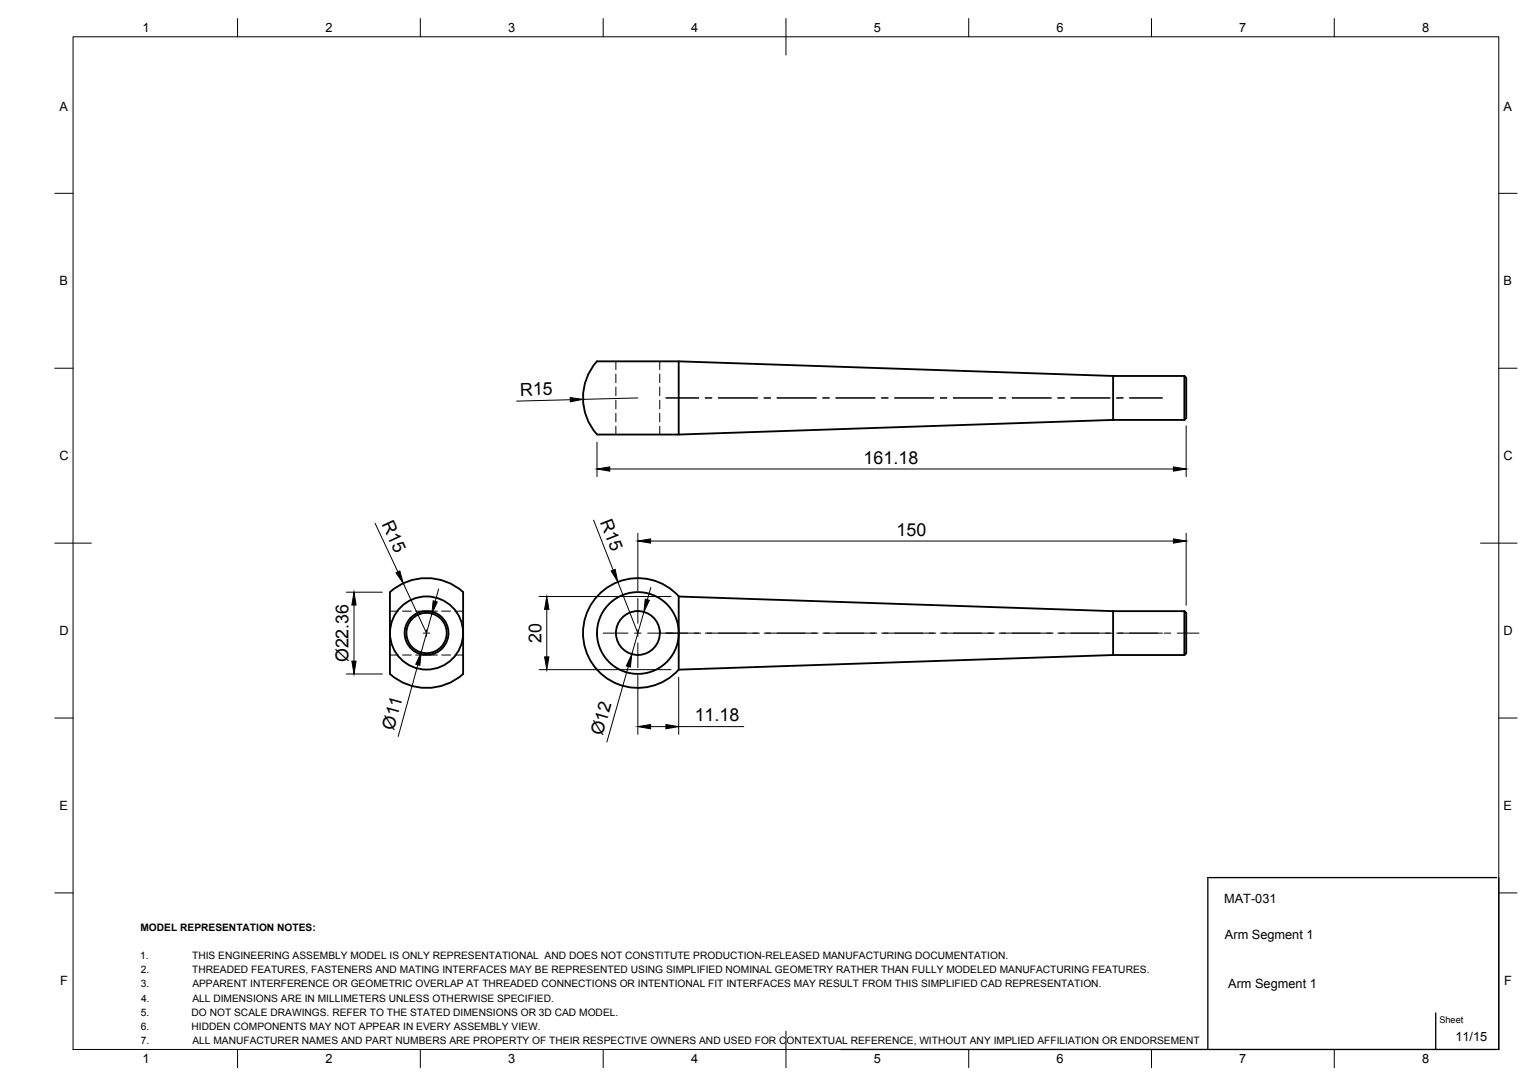
ISO-10303-21;
HEADER;
/* Generated by software containing ST-Developer
 * from STEP Tools, Inc. (www.steptools.com) 
 */

FILE_DESCRIPTION(
/* description */ ('STEP AP214'),
/* implementation_level */ '2;1');

FILE_NAME(
/* name */ 'Arm Segment 1.step',
/* time_stamp */ '2026-11-14T06:58:01-08:00',
/* author */ (''),
/* organization */ (''),
/* preprocessor_version */ 'ST-DEVELOPER v20.2',
/* originating_system */ 'Autodesk Translation Framework v15.17.0.0',
/* authorisation */ '');

FILE_SCHEMA (('AUTOMOTIVE_DESIGN { 1 0 10303 214 3 1 1 }'));
ENDSEC;

DATA;
#10=MECHANICAL_DESIGN_GEOMETRIC_PRESENTATION_REPRESENTATION('',(#1154),#38635);
#87=SPHERICAL_SURFACE('',#18128,15.);
#88=SPHERICAL_SURFACE('',#18136,15.);
#876=FACE_BOUND('',#2871,.T.);
#877=FACE_BOUND('',#2873,.T.);
#1027=CONICAL_SURFACE('',#18140,6.,0.0336517539394116);
#1028=CONICAL_SURFACE('',#18144,5.5,0.785398163397448);
#1120=SHAPE_REPRESENTATION_RELATIONSHIP('SRR','None',#38693,#1134);
#1134=ADVANCED_BREP_SHAPE_REPRESENTATION('',(#1180),#38629);
#1154=STYLED_ITEM('',(#38765),#1180);
#1180=MANIFOLD_SOLID_BREP('Body1',#17620);
#1260=PLANE('',#18146);
#1261=PLANE('',#18147);
#1262=PLANE('',#18148);
#1843=FACE_OUTER_BOUND('',#2863,.T.);
#1844=FACE_OUTER_BOUND('',#2864,.T.);
#1845=FACE_OUTER_BOUND('',#2865,.T.);
#1846=FACE_OUTER_BOUND('',#2866,.T.);
#1847=FACE_OUTER_BOUND('',#2867,.T.);
#1848=FACE_OUTER_BOUND('',#2868,.T.);
#1849=FACE_OUTER_BOUND('',#2869,.T.);
#1850=FACE_OUTER_BOUND('',#2870,.T.);
#1851=FACE_OUTER_BOUND('',#2872,.T.);
#2863=EDGE_LOOP('',(#11861,#11862,#11863,#11864));
#2864=EDGE_LOOP('',(#11865,#11866,#11867,#11868));
#2865=EDGE_LOOP('',(#11869,#11870,#11871,#11872));
#2866=EDGE_LOOP('',(#11873,#11874,#11875,#11876,#11877));
#2867=EDGE_LOOP('',(#11878,#11879,#11880,#11881));
#2868=EDGE_LOOP('',(#11882,#11883,#11884,#11885));
#2869=EDGE_LOOP('',(#11886));
#2870=EDGE_LOOP('',(#11887,#11888));
#2871=EDGE_LOOP('',(#11889));
#2872=EDGE_LOOP('',(#11890,#11891));
#2873=EDGE_LOOP('',(#11892));
#3897=LINE('',#32014,#4841);
#3898=LINE('',#32022,#4842);
#3899=LINE('',#32026,#4843);
#3900=LINE('',#32030,#4844);
#4841=VECTOR('',#20638,6.);
#4842=VECTOR('',#20651,6.);
#4843=VECTOR('',#20656,6.);
#4844=VECTOR('',#20661,5.5);
#5727=CIRCLE('',#18129,15.);
#5728=CIRCLE('',#18130,11.1803398874989);
#5729=CIRCLE('',#18131,10.);
#5730=CIRCLE('',#18132,11.1803398874989);
#5731=CIRCLE('',#18134,6.);
#5732=CIRCLE('',#18135,6.);
#5733=CIRCLE('',#18137,11.1803398874989);
#5734=CIRCLE('',#18138,10.);
#5735=CIRCLE('',#18139,11.1803398874989);
#5736=CIRCLE('',#18141,6.);
#5737=CIRCLE('',#18143,6.);
#5738=CIRCLE('',#18145,5.5);
#6820=VERTEX_POINT('',#32002);
#6821=VERTEX_POINT('',#32003);
#6822=VERTEX_POINT('',#32005);
#6823=VERTEX_POINT('',#32007);
#6824=VERTEX_POINT('',#32011);
#6825=VERTEX_POINT('',#32013);
#6826=VERTEX_POINT('',#32021);
#6827=VERTEX_POINT('',#32025);
#6828=VERTEX_POINT('',#32029);
#8717=EDGE_CURVE('',#6820,#6821,#5727,.T.);
#8718=EDGE_CURVE('',#6820,#6822,#5728,.T.);
#8719=EDGE_CURVE('',#6822,#6823,#5729,.T.);
#8720=EDGE_CURVE('',#6823,#6821,#5730,.T.);
#8721=EDGE_CURVE('',#6824,#6824,#5731,.T.);
#8722=EDGE_CURVE('',#6824,#6825,#3897,.T.);
#8723=EDGE_CURVE('',#6825,#6825,#5732,.T.);
#8724=EDGE_CURVE('',#6821,#6823,#5733,.T.);
#8725=EDGE_CURVE('',#6823,#6822,#5734,.T.);
#8726=EDGE_CURVE('',#6822,#6820,#5735,.T.);
#8727=EDGE_CURVE('',#6822,#6826,#3898,.T.);
#8728=EDGE_CURVE('',#6826,#6826,#5736,.T.);
#8729=EDGE_CURVE('',#6826,#6827,#3899,.T.);
#8730=EDGE_CURVE('',#6827,#6827,#5737,.T.);
#8731=EDGE_CURVE('',#6827,#6828,#3900,.T.);
#8732=EDGE_CURVE('',#6828,#6828,#5738,.T.);
#11861=ORIENTED_EDGE('',*,*,#8717,.F.);
#11862=ORIENTED_EDGE('',*,*,#8718,.T.);
#11863=ORIENTED_EDGE('',*,*,#8719,.T.);
#11864=ORIENTED_EDGE('',*,*,#8720,.T.);
#11865=ORIENTED_EDGE('',*,*,#8721,.F.);
#11866=ORIENTED_EDGE('',*,*,#8722,.T.);
#11867=ORIENTED_EDGE('',*,*,#8723,.T.);
#11868=ORIENTED_EDGE('',*,*,#8722,.F.);
#11869=ORIENTED_EDGE('',*,*,#8717,.T.);
#11870=ORIENTED_EDGE('',*,*,#8724,.T.);
#11871=ORIENTED_EDGE('',*,*,#8725,.T.);
#11872=ORIENTED_EDGE('',*,*,#8726,.T.);
#11873=ORIENTED_EDGE('',*,*,#8719,.F.);
#11874=ORIENTED_EDGE('',*,*,#8727,.T.);
#11875=ORIENTED_EDGE('',*,*,#8728,.T.);
#11876=ORIENTED_EDGE('',*,*,#8727,.F.);
#11877=ORIENTED_EDGE('',*,*,#8725,.F.);
#11878=ORIENTED_EDGE('',*,*,#8728,.F.);
#11879=ORIENTED_EDGE('',*,*,#8729,.T.);
#11880=ORIENTED_EDGE('',*,*,#8730,.T.);
#11881=ORIENTED_EDGE('',*,*,#8729,.F.);
#11882=ORIENTED_EDGE('',*,*,#8730,.F.);
#11883=ORIENTED_EDGE('',*,*,#8731,.T.);
#11884=ORIENTED_EDGE('',*,*,#8732,.T.);
#11885=ORIENTED_EDGE('',*,*,#8731,.F.);
#11886=ORIENTED_EDGE('',*,*,#8732,.F.);
#11887=ORIENTED_EDGE('',*,*,#8720,.F.);
#11888=ORIENTED_EDGE('',*,*,#8724,.F.);
#11889=ORIENTED_EDGE('',*,*,#8723,.F.);
#11890=ORIENTED_EDGE('',*,*,#8726,.F.);
#11891=ORIENTED_EDGE('',*,*,#8718,.F.);
#11892=ORIENTED_EDGE('',*,*,#8721,.T.);
#16339=CYLINDRICAL_SURFACE('',#18133,6.);
#16340=CYLINDRICAL_SURFACE('',#18142,6.);
#16802=ADVANCED_FACE('',(#1843),#87,.T.);
#16803=ADVANCED_FACE('',(#1844),#16339,.F.);
#16804=ADVANCED_FACE('',(#1845),#88,.T.);
#16805=ADVANCED_FACE('',(#1846),#1027,.T.);
#16806=ADVANCED_FACE('',(#1847),#16340,.T.);
#16807=ADVANCED_FACE('',(#1848),#1028,.T.);
#16808=ADVANCED_FACE('',(#1849),#1260,.F.);
#16809=ADVANCED_FACE('',(#1850,#876),#1261,.F.);
#16810=ADVANCED_FACE('',(#1851,#877),#1262,.F.);
#17620=CLOSED_SHELL('',(#16802,#16803,#16804,#16805,#16806,#16807,#16808,
#16809,#16810));
#18127=AXIS2_PLACEMENT_3D('',#32000,#20622,#20623);
#18128=AXIS2_PLACEMENT_3D('',#32001,#20624,#20625);
#18129=AXIS2_PLACEMENT_3D('',#32004,#20626,#20627);
#18130=AXIS2_PLACEMENT_3D('',#32006,#20628,#20629);
#18131=AXIS2_PLACEMENT_3D('',#32008,#20630,#20631);
#18132=AXIS2_PLACEMENT_3D('',#32009,#20632,#20633);
#18133=AXIS2_PLACEMENT_3D('',#32010,#20634,#20635);
#18134=AXIS2_PLACEMENT_3D('',#32012,#20636,#20637);
#18135=AXIS2_PLACEMENT_3D('',#32015,#20639,#20640);
#18136=AXIS2_PLACEMENT_3D('',#32016,#20641,#20642);
#18137=AXIS2_PLACEMENT_3D('',#32017,#20643,#20644);
#18138=AXIS2_PLACEMENT_3D('',#32018,#20645,#20646);
#18139=AXIS2_PLACEMENT_3D('',#32019,#20647,#20648);
#18140=AXIS2_PLACEMENT_3D('',#32020,#20649,#20650);
#18141=AXIS2_PLACEMENT_3D('',#32023,#20652,#20653);
#18142=AXIS2_PLACEMENT_3D('',#32024,#20654,#20655);
#18143=AXIS2_PLACEMENT_3D('',#32027,#20657,#20658);
#18144=AXIS2_PLACEMENT_3D('',#32028,#20659,#20660);
#18145=AXIS2_PLACEMENT_3D('',#32031,#20662,#20663);
#18146=AXIS2_PLACEMENT_3D('',#32032,#20664,#20665);
#18147=AXIS2_PLACEMENT_3D('',#32033,#20666,#20667);
#18148=AXIS2_PLACEMENT_3D('',#32034,#20668,#20669);
#20622=DIRECTION('axis',(0.,0.,1.));
#20623=DIRECTION('refdir',(1.,0.,0.));
#20624=DIRECTION('center_axis',(0.,6.12323399573677E-17,-1.));
#20625=DIRECTION('ref_axis',(0.,1.,0.));
#20626=DIRECTION('center_axis',(-1.,1.22464679914735E-16,0.));
#20627=DIRECTION('ref_axis',(-1.22464679914735E-16,-1.,0.));
#20628=DIRECTION('center_axis',(0.,0.,1.));
#20629=DIRECTION('ref_axis',(1.,0.,0.));
#20630=DIRECTION('center_axis',(-1.,0.,0.));
#20631=DIRECTION('ref_axis',(0.,0.,1.));
#20632=DIRECTION('center_axis',(0.,0.,-1.));
#20633=DIRECTION('ref_axis',(-1.,0.,0.));
#20634=DIRECTION('center_axis',(0.,0.,1.));
#20635=DIRECTION('ref_axis',(1.,0.,0.));
#20636=DIRECTION('center_axis',(0.,0.,1.));
#20637=DIRECTION('ref_axis',(1.,0.,0.));
#20638=DIRECTION('',(0.,0.,1.));
#20639=DIRECTION('center_axis',(0.,0.,1.));
#20640=DIRECTION('ref_axis',(1.,0.,0.));
#20641=DIRECTION('center_axis',(0.,6.12323399573677E-17,-1.));
#20642=DIRECTION('ref_axis',(0.,1.,0.));
#20643=DIRECTION('center_axis',(0.,0.,-1.));
#20644=DIRECTION('ref_axis',(-1.,0.,0.));
#20645=DIRECTION('center_axis',(-1.,0.,0.));
#20646=DIRECTION('ref_axis',(0.,0.,1.));
#20647=DIRECTION('center_axis',(0.,0.,1.));
#20648=DIRECTION('ref_axis',(1.,0.,0.));
#20649=DIRECTION('center_axis',(-1.,0.,0.));
#20650=DIRECTION('ref_axis',(0.,0.,1.));
#20651=DIRECTION('',(0.999433833160616,4.1203734923357E-18,0.033645402863948));
#20652=DIRECTION('center_axis',(-1.,0.,0.));
#20653=DIRECTION('ref_axis',(0.,0.,1.));
#20654=DIRECTION('center_axis',(-1.,0.,0.));
#20655=DIRECTION('ref_axis',(0.,0.,1.));
#20656=DIRECTION('',(1.,0.,0.));
#20657=DIRECTION('center_axis',(-1.,0.,0.));
#20658=DIRECTION('ref_axis',(0.,0.,1.));
#20659=DIRECTION('center_axis',(-1.,0.,0.));
#20660=DIRECTION('ref_axis',(0.,0.,1.));
#20661=DIRECTION('',(0.707106781186548,8.65956056235493E-17,0.707106781186547));
#20662=DIRECTION('center_axis',(-1.,0.,0.));
#20663=DIRECTION('ref_axis',(0.,0.,1.));
#20664=DIRECTION('center_axis',(-1.,0.,0.));
#20665=DIRECTION('ref_axis',(0.,0.,1.));
#20666=DIRECTION('center_axis',(0.,0.,-1.));
#20667=DIRECTION('ref_axis',(-1.,0.,0.));
#20668=DIRECTION('center_axis',(0.,0.,1.));
#20669=DIRECTION('ref_axis',(1.,0.,0.));
#32000=CARTESIAN_POINT('',(0.,0.,0.));
#32001=CARTESIAN_POINT('Origin',(0.,0.,0.));
#32002=CARTESIAN_POINT('',(-1.36919674566051E-15,-11.1803398874989,-10.));
#32003=CARTESIAN_POINT('',(-1.36919674566051E-15,-11.1803398874989,10.));
#32004=CARTESIAN_POINT('Origin',(0.,0.,0.));
#32005=CARTESIAN_POINT('',(11.1803398874989,0.,-10.));
#32006=CARTESIAN_POINT('Origin',(0.,0.,-10.));
#32007=CARTESIAN_POINT('',(11.1803398874989,0.,10.));
#32008=CARTESIAN_POINT('Origin',(11.1803398874989,0.,0.));
#32009=CARTESIAN_POINT('Origin',(0.,0.,10.));
#32010=CARTESIAN_POINT('Origin',(0.,0.,-10.));
#32011=CARTESIAN_POINT('',(-6.,-7.34788079488412E-16,-10.));
#32012=CARTESIAN_POINT('Origin',(0.,0.,-10.));
#32013=CARTESIAN_POINT('',(-6.,-7.34788079488412E-16,10.));
#32014=CARTESIAN_POINT('',(-6.,-7.34788079488412E-16,-10.));
#32015=CARTESIAN_POINT('Origin',(0.,0.,10.));
#32016=CARTESIAN_POINT('Origin',(0.,0.,0.));
#32017=CARTESIAN_POINT('Origin',(0.,0.,10.));
#32018=CARTESIAN_POINT('Origin',(11.1803398874989,0.,0.));
#32019=CARTESIAN_POINT('Origin',(0.,0.,-10.));
#32020=CARTESIAN_POINT('Origin',(130.,0.,0.));
#32021=CARTESIAN_POINT('',(130.,-7.34788079488412E-16,-6.));
#32022=CARTESIAN_POINT('',(130.,-7.34788079488412E-16,-6.));
#32023=CARTESIAN_POINT('Origin',(130.,0.,0.));
#32024=CARTESIAN_POINT('Origin',(-71.1905382258649,0.,0.));
#32025=CARTESIAN_POINT('',(149.5,-7.34788079488412E-16,-6.));
#32026=CARTESIAN_POINT('',(-71.1905382258649,-7.34788079488412E-16,-6.));
#32027=CARTESIAN_POINT('Origin',(149.5,0.,0.));
#32028=CARTESIAN_POINT('Origin',(150.,0.,0.));
#32029=CARTESIAN_POINT('',(150.,-6.73555739531044E-16,-5.5));
#32030=CARTESIAN_POINT('',(150.,-6.73555739531044E-16,-5.5));
#32031=CARTESIAN_POINT('Origin',(150.,0.,0.));
#32032=CARTESIAN_POINT('Origin',(150.,0.,0.));
#32033=CARTESIAN_POINT('Origin',(11.1803398874989,-15.,10.));
#32034=CARTESIAN_POINT('Origin',(11.1803398874989,-15.,-10.));
#38613=UNCERTAINTY_MEASURE_WITH_UNIT(LENGTH_MEASURE(0.01),#38636,
'DISTANCE_ACCURACY_VALUE',
'Maximum model space distance between geometric entities at asserted c
onnectivities');
#38619=UNCERTAINTY_MEASURE_WITH_UNIT(LENGTH_MEASURE(0.01),#38636,
'DISTANCE_ACCURACY_VALUE',
'Maximum model space distance between geometric entities at asserted c
onnectivities');
#38629=(
GEOMETRIC_REPRESENTATION_CONTEXT(3)
GLOBAL_UNCERTAINTY_ASSIGNED_CONTEXT((#38613))
GLOBAL_UNIT_ASSIGNED_CONTEXT((#38636,#38638,#38639))
REPRESENTATION_CONTEXT('','3D')
);
#38635=(
GEOMETRIC_REPRESENTATION_CONTEXT(3)
GLOBAL_UNCERTAINTY_ASSIGNED_CONTEXT((#38619))
GLOBAL_UNIT_ASSIGNED_CONTEXT((#38636,#38638,#38639))
REPRESENTATION_CONTEXT('','3D')
);
#38636=(
LENGTH_UNIT()
NAMED_UNIT(*)
SI_UNIT(.MILLI.,.METRE.)
);
#38638=(
NAMED_UNIT(*)
PLANE_ANGLE_UNIT()
SI_UNIT($,.RADIAN.)
);
#38639=(
NAMED_UNIT(*)
SI_UNIT($,.STERADIAN.)
SOLID_ANGLE_UNIT()
);
#38649=SHAPE_DEFINITION_REPRESENTATION(#38664,#38693);
#38664=PRODUCT_DEFINITION_SHAPE('',$,#38709);
#38693=SHAPE_REPRESENTATION('',(#18127),#38629);
#38699=PRODUCT_DEFINITION_CONTEXT('part definition',#38746,'design');
#38709=PRODUCT_DEFINITION('Arm Segment 1','Arm Segment 1',#38724,#38699);
#38724=PRODUCT_DEFINITION_FORMATION('',$,#38757);
#38746=APPLICATION_CONTEXT(
'Core Data for Automotive Mechanical Design Process');
#38747=PRODUCT_CONTEXT('part definition',#38746,'mechanical');
#38757=PRODUCT('Arm Segment 1','Arm Segment 1',$,(#38747));
#38765=PRESENTATION_STYLE_ASSIGNMENT((#38772));
#38772=SURFACE_STYLE_USAGE(.BOTH.,#38779);
#38779=SURFACE_SIDE_STYLE('',(#38786));
#38786=SURFACE_STYLE_FILL_AREA(#38793);
#38793=FILL_AREA_STYLE('Opaque(227,224,212)',(#38800));
#38800=FILL_AREA_STYLE_COLOUR('Opaque(227,224,212)',#38807);
#38807=COLOUR_RGB('Opaque(227,224,212)',0.890196078431372,0.87843137254902,
0.831372549019608);
ENDSEC;
END-ISO-10303-21;
